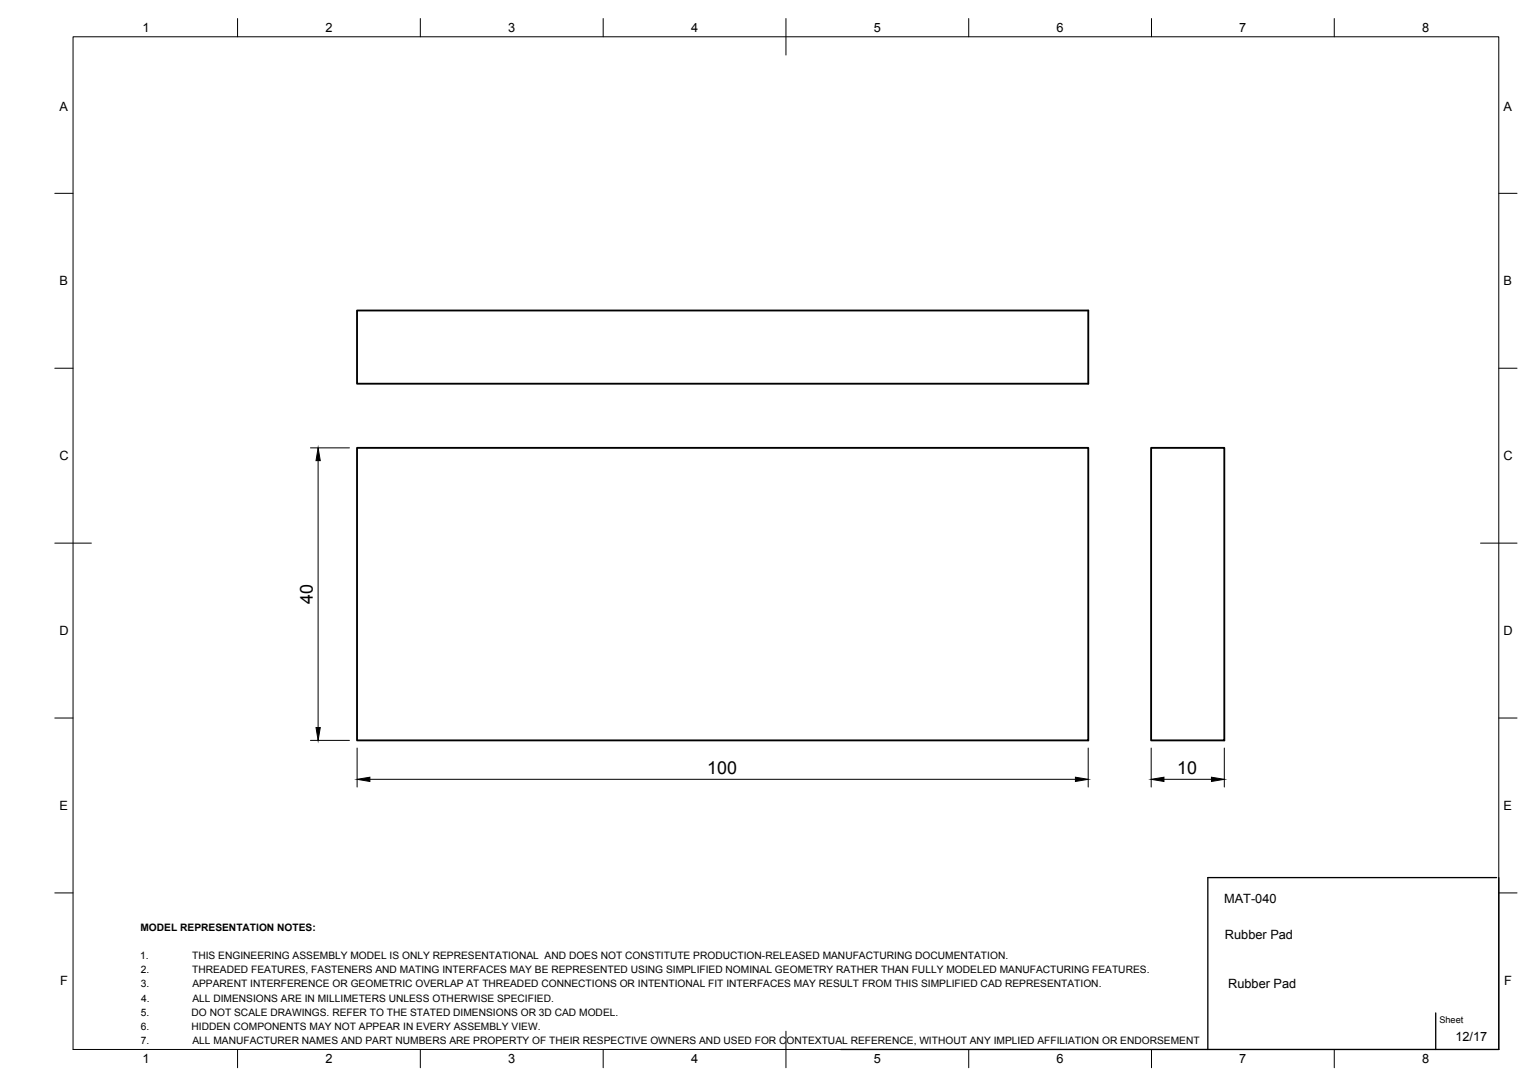
ISO-10303-21;
HEADER;
/* Generated by software containing ST-Developer
 * from STEP Tools, Inc. (www.steptools.com) 
 */

FILE_DESCRIPTION(
/* description */ ('STEP AP214'),
/* implementation_level */ '2;1');

FILE_NAME(
/* name */ 'Rubber Pad.step',
/* time_stamp */ '2026-11-14T21:53:28-08:00',
/* author */ (''),
/* organization */ (''),
/* preprocessor_version */ 'ST-DEVELOPER v20.2',
/* originating_system */ 'Autodesk Translation Framework v15.17.0.0',
/* authorisation */ '');

FILE_SCHEMA (('AUTOMOTIVE_DESIGN { 1 0 10303 214 3 1 1 }'));
ENDSEC;

DATA;
#10=MECHANICAL_DESIGN_GEOMETRIC_PRESENTATION_REPRESENTATION('',(#331),#20176);
#299=SHAPE_REPRESENTATION_RELATIONSHIP('SRR','None',#20262,#311);
#311=ADVANCED_BREP_SHAPE_REPRESENTATION('',(#358),#20168);
#331=STYLED_ITEM('',(#20337),#358);
#358=MANIFOLD_SOLID_BREP('Body1',#10949);
#840=PLANE('',#11957);
#841=PLANE('',#11958);
#842=PLANE('',#11959);
#843=PLANE('',#11960);
#844=PLANE('',#11961);
#845=PLANE('',#11962);
#1378=FACE_OUTER_BOUND('',#2136,.T.);
#1379=FACE_OUTER_BOUND('',#2137,.T.);
#1380=FACE_OUTER_BOUND('',#2138,.T.);
#1381=FACE_OUTER_BOUND('',#2139,.T.);
#1382=FACE_OUTER_BOUND('',#2140,.T.);
#1383=FACE_OUTER_BOUND('',#2141,.T.);
#2136=EDGE_LOOP('',(#9693,#9694,#9695,#9696));
#2137=EDGE_LOOP('',(#9697,#9698,#9699,#9700));
#2138=EDGE_LOOP('',(#9701,#9702,#9703,#9704));
#2139=EDGE_LOOP('',(#9705,#9706,#9707,#9708));
#2140=EDGE_LOOP('',(#9709,#9710,#9711,#9712));
#2141=EDGE_LOOP('',(#9713,#9714,#9715,#9716));
#3134=LINE('',#19597,#4122);
#3135=LINE('',#19599,#4123);
#3136=LINE('',#19601,#4124);
#3137=LINE('',#19602,#4125);
#3138=LINE('',#19605,#4126);
#3139=LINE('',#19607,#4127);
#3140=LINE('',#19608,#4128);
#3141=LINE('',#19611,#4129);
#3142=LINE('',#19613,#4130);
#3143=LINE('',#19614,#4131);
#3144=LINE('',#19616,#4132);
#3145=LINE('',#19617,#4133);
#4122=VECTOR('',#14776,1000.);
#4123=VECTOR('',#14777,1000.);
#4124=VECTOR('',#14778,1000.);
#4125=VECTOR('',#14779,1000.);
#4126=VECTOR('',#14782,1000.);
#4127=VECTOR('',#14783,1000.);
#4128=VECTOR('',#14784,1000.);
#4129=VECTOR('',#14787,1000.);
#4130=VECTOR('',#14788,1000.);
#4131=VECTOR('',#14789,1000.);
#4132=VECTOR('',#14792,1000.);
#4133=VECTOR('',#14793,1000.);
#5534=VERTEX_POINT('',#19595);
#5535=VERTEX_POINT('',#19596);
#5536=VERTEX_POINT('',#19598);
#5537=VERTEX_POINT('',#19600);
#5538=VERTEX_POINT('',#19604);
#5539=VERTEX_POINT('',#19606);
#5540=VERTEX_POINT('',#19610);
#5541=VERTEX_POINT('',#19612);
#6957=EDGE_CURVE('',#5534,#5535,#3134,.T.);
#6958=EDGE_CURVE('',#5536,#5535,#3135,.T.);
#6959=EDGE_CURVE('',#5537,#5536,#3136,.T.);
#6960=EDGE_CURVE('',#5537,#5534,#3137,.T.);
#6961=EDGE_CURVE('',#5535,#5538,#3138,.T.);
#6962=EDGE_CURVE('',#5539,#5538,#3139,.T.);
#6963=EDGE_CURVE('',#5536,#5539,#3140,.T.);
#6964=EDGE_CURVE('',#5538,#5540,#3141,.T.);
#6965=EDGE_CURVE('',#5541,#5540,#3142,.T.);
#6966=EDGE_CURVE('',#5539,#5541,#3143,.T.);
#6967=EDGE_CURVE('',#5540,#5534,#3144,.T.);
#6968=EDGE_CURVE('',#5541,#5537,#3145,.T.);
#9693=ORIENTED_EDGE('',*,*,#6957,.T.);
#9694=ORIENTED_EDGE('',*,*,#6958,.F.);
#9695=ORIENTED_EDGE('',*,*,#6959,.F.);
#9696=ORIENTED_EDGE('',*,*,#6960,.T.);
#9697=ORIENTED_EDGE('',*,*,#6961,.T.);
#9698=ORIENTED_EDGE('',*,*,#6962,.F.);
#9699=ORIENTED_EDGE('',*,*,#6963,.F.);
#9700=ORIENTED_EDGE('',*,*,#6958,.T.);
#9701=ORIENTED_EDGE('',*,*,#6964,.T.);
#9702=ORIENTED_EDGE('',*,*,#6965,.F.);
#9703=ORIENTED_EDGE('',*,*,#6966,.F.);
#9704=ORIENTED_EDGE('',*,*,#6962,.T.);
#9705=ORIENTED_EDGE('',*,*,#6967,.T.);
#9706=ORIENTED_EDGE('',*,*,#6960,.F.);
#9707=ORIENTED_EDGE('',*,*,#6968,.F.);
#9708=ORIENTED_EDGE('',*,*,#6965,.T.);
#9709=ORIENTED_EDGE('',*,*,#6959,.T.);
#9710=ORIENTED_EDGE('',*,*,#6963,.T.);
#9711=ORIENTED_EDGE('',*,*,#6966,.T.);
#9712=ORIENTED_EDGE('',*,*,#6968,.T.);
#9713=ORIENTED_EDGE('',*,*,#6957,.F.);
#9714=ORIENTED_EDGE('',*,*,#6967,.F.);
#9715=ORIENTED_EDGE('',*,*,#6964,.F.);
#9716=ORIENTED_EDGE('',*,*,#6961,.F.);
#10830=ADVANCED_FACE('',(#1378),#840,.F.);
#10831=ADVANCED_FACE('',(#1379),#841,.F.);
#10832=ADVANCED_FACE('',(#1380),#842,.F.);
#10833=ADVANCED_FACE('',(#1381),#843,.F.);
#10834=ADVANCED_FACE('',(#1382),#844,.T.);
#10835=ADVANCED_FACE('',(#1383),#845,.F.);
#10949=CLOSED_SHELL('',(#10830,#10831,#10832,#10833,#10834,#10835));
#11956=AXIS2_PLACEMENT_3D('',#19593,#14772,#14773);
#11957=AXIS2_PLACEMENT_3D('',#19594,#14774,#14775);
#11958=AXIS2_PLACEMENT_3D('',#19603,#14780,#14781);
#11959=AXIS2_PLACEMENT_3D('',#19609,#14785,#14786);
#11960=AXIS2_PLACEMENT_3D('',#19615,#14790,#14791);
#11961=AXIS2_PLACEMENT_3D('',#19618,#14794,#14795);
#11962=AXIS2_PLACEMENT_3D('',#19619,#14796,#14797);
#14772=DIRECTION('axis',(0.,0.,1.));
#14773=DIRECTION('refdir',(1.,0.,0.));
#14774=DIRECTION('center_axis',(-1.,0.,0.));
#14775=DIRECTION('ref_axis',(0.,0.,1.));
#14776=DIRECTION('',(0.,1.,0.));
#14777=DIRECTION('',(0.,0.,-1.));
#14778=DIRECTION('',(0.,1.,0.));
#14779=DIRECTION('',(0.,0.,-1.));
#14780=DIRECTION('center_axis',(0.,-1.,0.));
#14781=DIRECTION('ref_axis',(0.,0.,-1.));
#14782=DIRECTION('',(-1.,0.,0.));
#14783=DIRECTION('',(0.,0.,-1.));
#14784=DIRECTION('',(-1.,0.,0.));
#14785=DIRECTION('center_axis',(1.,3.46944695195361E-16,0.));
#14786=DIRECTION('ref_axis',(-3.46944695195361E-16,1.,0.));
#14787=DIRECTION('',(3.46944695195361E-16,-1.,0.));
#14788=DIRECTION('',(0.,0.,-1.));
#14789=DIRECTION('',(3.46944695195361E-16,-1.,0.));
#14790=DIRECTION('center_axis',(0.,1.,0.));
#14791=DIRECTION('ref_axis',(0.,0.,1.));
#14792=DIRECTION('',(1.,0.,0.));
#14793=DIRECTION('',(1.,0.,0.));
#14794=DIRECTION('center_axis',(0.,0.,1.));
#14795=DIRECTION('ref_axis',(1.,0.,0.));
#14796=DIRECTION('center_axis',(0.,0.,1.));
#14797=DIRECTION('ref_axis',(1.,0.,0.));
#19593=CARTESIAN_POINT('',(0.,0.,0.));
#19594=CARTESIAN_POINT('Origin',(50.,20.,10.));
#19595=CARTESIAN_POINT('',(50.,-20.,0.));
#19596=CARTESIAN_POINT('',(50.,20.,0.));
#19597=CARTESIAN_POINT('',(50.,20.,0.));
#19598=CARTESIAN_POINT('',(50.,20.,10.));
#19599=CARTESIAN_POINT('',(50.,20.,10.));
#19600=CARTESIAN_POINT('',(50.,-20.,10.));
#19601=CARTESIAN_POINT('',(50.,20.,10.));
#19602=CARTESIAN_POINT('',(50.,-20.,10.));
#19603=CARTESIAN_POINT('Origin',(-50.,20.,10.));
#19604=CARTESIAN_POINT('',(-50.,20.,0.));
#19605=CARTESIAN_POINT('',(-50.,20.,0.));
#19606=CARTESIAN_POINT('',(-50.,20.,10.));
#19607=CARTESIAN_POINT('',(-50.,20.,10.));
#19608=CARTESIAN_POINT('',(-50.,20.,10.));
#19609=CARTESIAN_POINT('Origin',(-50.,20.,10.));
#19610=CARTESIAN_POINT('',(-50.,-20.,0.));
#19611=CARTESIAN_POINT('',(-50.,20.,0.));
#19612=CARTESIAN_POINT('',(-50.,-20.,10.));
#19613=CARTESIAN_POINT('',(-50.,-20.,10.));
#19614=CARTESIAN_POINT('',(-50.,20.,10.));
#19615=CARTESIAN_POINT('Origin',(-50.,-20.,10.));
#19616=CARTESIAN_POINT('',(-50.,-20.,0.));
#19617=CARTESIAN_POINT('',(-50.,-20.,10.));
#19618=CARTESIAN_POINT('Origin',(0.,0.,10.));
#19619=CARTESIAN_POINT('Origin',(0.,0.,0.));
#20152=UNCERTAINTY_MEASURE_WITH_UNIT(LENGTH_MEASURE(0.01),#20177,
'DISTANCE_ACCURACY_VALUE',
'Maximum model space distance between geometric entities at asserted c
onnectivities');
#20160=UNCERTAINTY_MEASURE_WITH_UNIT(LENGTH_MEASURE(0.01),#20177,
'DISTANCE_ACCURACY_VALUE',
'Maximum model space distance between geometric entities at asserted c
onnectivities');
#20168=(
GEOMETRIC_REPRESENTATION_CONTEXT(3)
GLOBAL_UNCERTAINTY_ASSIGNED_CONTEXT((#20152))
GLOBAL_UNIT_ASSIGNED_CONTEXT((#20177,#20179,#20180))
REPRESENTATION_CONTEXT('','3D')
);
#20176=(
GEOMETRIC_REPRESENTATION_CONTEXT(3)
GLOBAL_UNCERTAINTY_ASSIGNED_CONTEXT((#20160))
GLOBAL_UNIT_ASSIGNED_CONTEXT((#20177,#20179,#20180))
REPRESENTATION_CONTEXT('','3D')
);
#20177=(
LENGTH_UNIT()
NAMED_UNIT(*)
SI_UNIT(.MILLI.,.METRE.)
);
#20179=(
NAMED_UNIT(*)
PLANE_ANGLE_UNIT()
SI_UNIT($,.RADIAN.)
);
#20180=(
NAMED_UNIT(*)
SI_UNIT($,.STERADIAN.)
SOLID_ANGLE_UNIT()
);
#20188=SHAPE_DEFINITION_REPRESENTATION(#20203,#20262);
#20203=PRODUCT_DEFINITION_SHAPE('',$,#20278);
#20262=SHAPE_REPRESENTATION('',(#11956),#20168);
#20270=PRODUCT_DEFINITION_CONTEXT('part definition',#20317,'design');
#20278=PRODUCT_DEFINITION('Rubber Pad','Rubber Pad',#20293,#20270);
#20293=PRODUCT_DEFINITION_FORMATION('',$,#20326);
#20317=APPLICATION_CONTEXT(
'Core Data for Automotive Mechanical Design Process');
#20318=PRODUCT_CONTEXT('part definition',#20317,'mechanical');
#20326=PRODUCT('Rubber Pad','Rubber Pad',$,(#20318));
#20337=PRESENTATION_STYLE_ASSIGNMENT((#20342));
#20342=SURFACE_STYLE_USAGE(.BOTH.,#20347);
#20347=SURFACE_SIDE_STYLE('',(#20352));
#20352=SURFACE_STYLE_FILL_AREA(#20357);
#20357=FILL_AREA_STYLE('Opaque(31,36,43)',(#20362));
#20362=FILL_AREA_STYLE_COLOUR('Opaque(31,36,43)',#20367);
#20367=COLOUR_RGB('Opaque(31,36,43)',0.12156862745098,0.141176470588235,
0.168627450980392);
ENDSEC;
END-ISO-10303-21;
